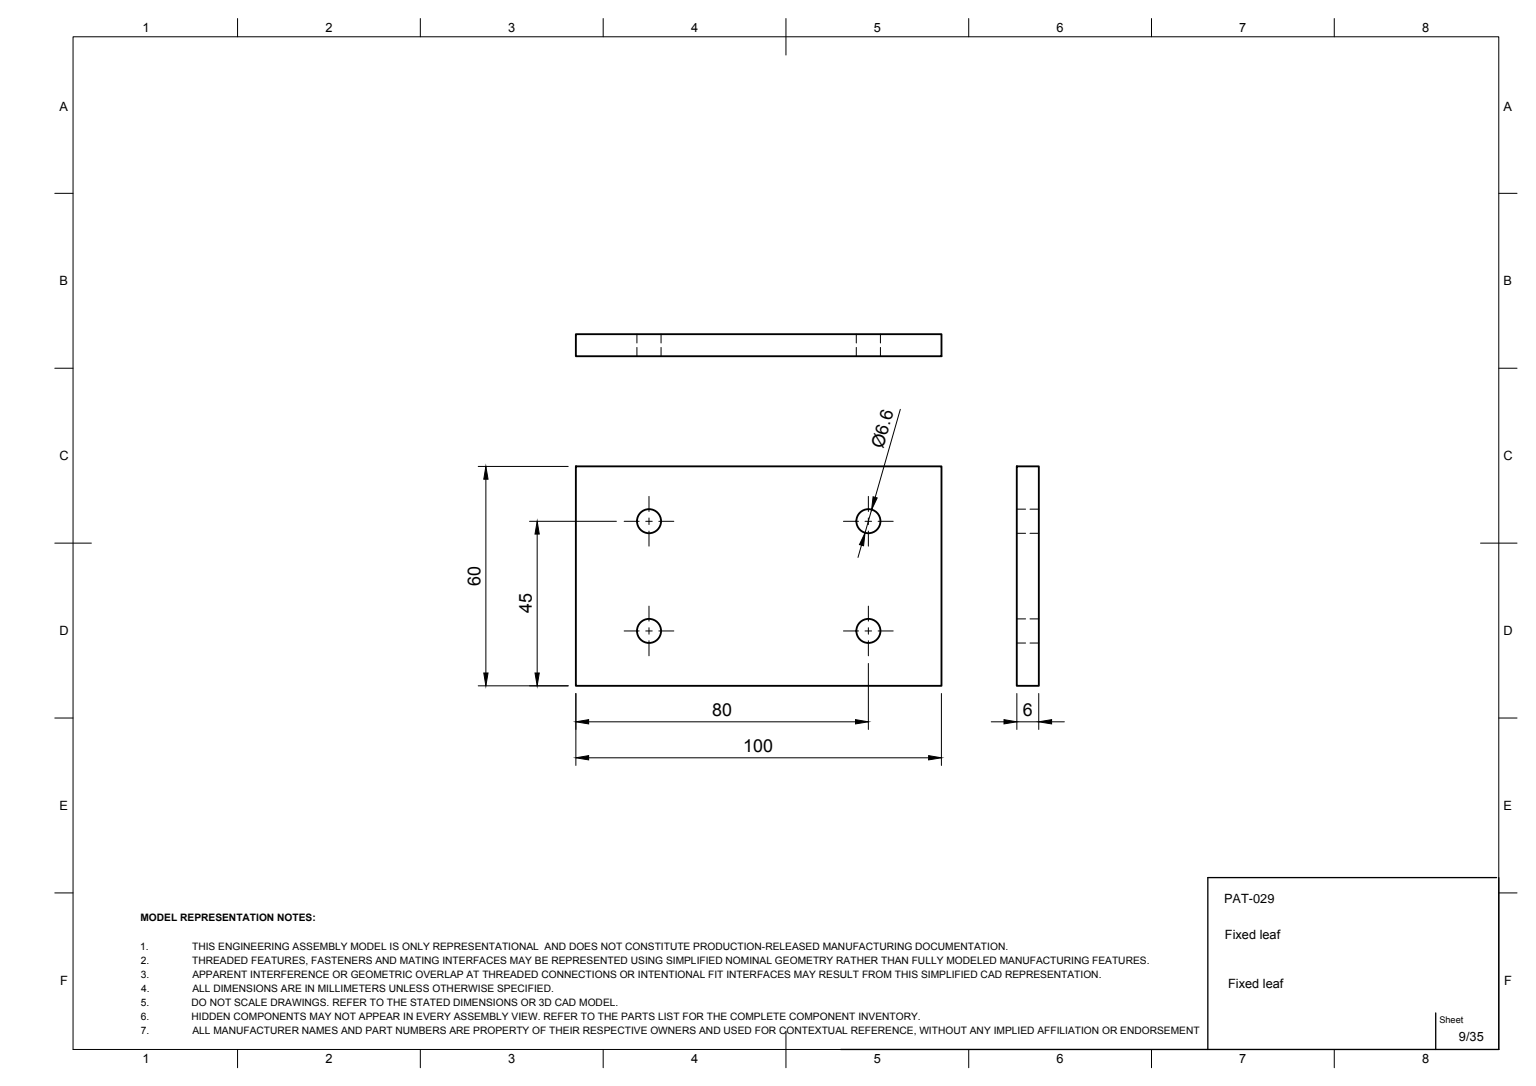
ISO-10303-21;
HEADER;
/* Generated by software containing ST-Developer
 * from STEP Tools, Inc. (www.steptools.com) 
 */

FILE_DESCRIPTION(
/* description */ ('Door-style hinge test fixture with detent'),
/* implementation_level */ '2;1');

FILE_NAME(
/* name */ 'Fixed leaf.step',
/* time_stamp */ '2026-10-28T03:24:57-07:00',
/* author */ (''),
/* organization */ (''),
/* preprocessor_version */ 'ST-DEVELOPER v20.2',
/* originating_system */ 'Autodesk Translation Framework v15.17.0.0',
/* authorisation */ '');

FILE_SCHEMA (('AUTOMOTIVE_DESIGN { 1 0 10303 214 3 1 1 }'));
ENDSEC;

DATA;
#10=MECHANICAL_DESIGN_GEOMETRIC_PRESENTATION_REPRESENTATION('',(#327),#9813);
#264=SHAPE_REPRESENTATION_RELATIONSHIP('SRR','None',#9941,#295);
#295=ADVANCED_BREP_SHAPE_REPRESENTATION('',(#367),#9784);
#327=STYLED_ITEM('',(#10176),#367);
#367=MANIFOLD_SOLID_BREP('Body1',#4758);
#415=FACE_BOUND('',#1007,.T.);
#416=FACE_BOUND('',#1008,.T.);
#417=FACE_BOUND('',#1009,.T.);
#418=FACE_BOUND('',#1010,.T.);
#419=FACE_BOUND('',#1013,.T.);
#420=FACE_BOUND('',#1014,.T.);
#421=FACE_BOUND('',#1015,.T.);
#422=FACE_BOUND('',#1016,.T.);
#530=PLANE('',#5211);
#531=PLANE('',#5212);
#532=PLANE('',#5213);
#533=PLANE('',#5214);
#534=PLANE('',#5215);
#535=PLANE('',#5216);
#701=FACE_OUTER_BOUND('',#1002,.T.);
#702=FACE_OUTER_BOUND('',#1003,.T.);
#703=FACE_OUTER_BOUND('',#1004,.T.);
#704=FACE_OUTER_BOUND('',#1005,.T.);
#705=FACE_OUTER_BOUND('',#1006,.T.);
#706=FACE_OUTER_BOUND('',#1011,.T.);
#707=FACE_OUTER_BOUND('',#1012,.T.);
#708=FACE_OUTER_BOUND('',#1017,.T.);
#709=FACE_OUTER_BOUND('',#1018,.T.);
#710=FACE_OUTER_BOUND('',#1019,.T.);
#1002=EDGE_LOOP('',(#3375,#3376,#3377,#3378));
#1003=EDGE_LOOP('',(#3379,#3380,#3381,#3382));
#1004=EDGE_LOOP('',(#3383,#3384,#3385,#3386));
#1005=EDGE_LOOP('',(#3387,#3388,#3389,#3390));
#1006=EDGE_LOOP('',(#3391,#3392,#3393,#3394));
#1007=EDGE_LOOP('',(#3395));
#1008=EDGE_LOOP('',(#3396));
#1009=EDGE_LOOP('',(#3397));
#1010=EDGE_LOOP('',(#3398));
#1011=EDGE_LOOP('',(#3399,#3400,#3401,#3402));
#1012=EDGE_LOOP('',(#3403,#3404,#3405,#3406));
#1013=EDGE_LOOP('',(#3407));
#1014=EDGE_LOOP('',(#3408));
#1015=EDGE_LOOP('',(#3409));
#1016=EDGE_LOOP('',(#3410));
#1017=EDGE_LOOP('',(#3411,#3412,#3413,#3414));
#1018=EDGE_LOOP('',(#3415,#3416,#3417,#3418));
#1019=EDGE_LOOP('',(#3419,#3420,#3421,#3422));
#1402=LINE('',#7486,#1722);
#1403=LINE('',#7492,#1723);
#1404=LINE('',#7498,#1724);
#1405=LINE('',#7504,#1725);
#1406=LINE('',#7509,#1726);
#1407=LINE('',#7511,#1727);
#1408=LINE('',#7513,#1728);
#1409=LINE('',#7514,#1729);
#1410=LINE('',#7517,#1730);
#1411=LINE('',#7519,#1731);
#1412=LINE('',#7520,#1732);
#1413=LINE('',#7523,#1733);
#1414=LINE('',#7525,#1734);
#1415=LINE('',#7526,#1735);
#1416=LINE('',#7528,#1736);
#1417=LINE('',#7529,#1737);
#1722=VECTOR('',#5945,0.33);
#1723=VECTOR('',#5952,0.33);
#1724=VECTOR('',#5959,0.33);
#1725=VECTOR('',#5966,0.33);
#1726=VECTOR('',#5971,1.);
#1727=VECTOR('',#5972,1.);
#1728=VECTOR('',#5973,1.);
#1729=VECTOR('',#5974,1.);
#1730=VECTOR('',#5977,1.);
#1731=VECTOR('',#5978,1.);
#1732=VECTOR('',#5979,1.);
#1733=VECTOR('',#5982,1.);
#1734=VECTOR('',#5983,1.);
#1735=VECTOR('',#5984,1.);
#1736=VECTOR('',#5987,1.);
#1737=VECTOR('',#5988,1.);
#1990=CIRCLE('',#5200,0.33);
#1991=CIRCLE('',#5201,0.33);
#1992=CIRCLE('',#5203,0.33);
#1993=CIRCLE('',#5204,0.33);
#1994=CIRCLE('',#5206,0.33);
#1995=CIRCLE('',#5207,0.33);
#1996=CIRCLE('',#5209,0.33);
#1997=CIRCLE('',#5210,0.33);
#2277=VERTEX_POINT('',#7483);
#2278=VERTEX_POINT('',#7485);
#2279=VERTEX_POINT('',#7489);
#2280=VERTEX_POINT('',#7491);
#2281=VERTEX_POINT('',#7495);
#2282=VERTEX_POINT('',#7497);
#2283=VERTEX_POINT('',#7501);
#2284=VERTEX_POINT('',#7503);
#2285=VERTEX_POINT('',#7507);
#2286=VERTEX_POINT('',#7508);
#2287=VERTEX_POINT('',#7510);
#2288=VERTEX_POINT('',#7512);
#2289=VERTEX_POINT('',#7516);
#2290=VERTEX_POINT('',#7518);
#2291=VERTEX_POINT('',#7522);
#2292=VERTEX_POINT('',#7524);
#2704=EDGE_CURVE('',#2277,#2277,#1990,.T.);
#2705=EDGE_CURVE('',#2277,#2278,#1402,.T.);
#2706=EDGE_CURVE('',#2278,#2278,#1991,.T.);
#2707=EDGE_CURVE('',#2279,#2279,#1992,.T.);
#2708=EDGE_CURVE('',#2279,#2280,#1403,.T.);
#2709=EDGE_CURVE('',#2280,#2280,#1993,.T.);
#2710=EDGE_CURVE('',#2281,#2281,#1994,.T.);
#2711=EDGE_CURVE('',#2281,#2282,#1404,.T.);
#2712=EDGE_CURVE('',#2282,#2282,#1995,.T.);
#2713=EDGE_CURVE('',#2283,#2283,#1996,.T.);
#2714=EDGE_CURVE('',#2283,#2284,#1405,.T.);
#2715=EDGE_CURVE('',#2284,#2284,#1997,.T.);
#2716=EDGE_CURVE('',#2285,#2286,#1406,.T.);
#2717=EDGE_CURVE('',#2286,#2287,#1407,.T.);
#2718=EDGE_CURVE('',#2288,#2287,#1408,.T.);
#2719=EDGE_CURVE('',#2285,#2288,#1409,.T.);
#2720=EDGE_CURVE('',#2289,#2285,#1410,.T.);
#2721=EDGE_CURVE('',#2290,#2288,#1411,.T.);
#2722=EDGE_CURVE('',#2289,#2290,#1412,.T.);
#2723=EDGE_CURVE('',#2291,#2289,#1413,.T.);
#2724=EDGE_CURVE('',#2292,#2290,#1414,.T.);
#2725=EDGE_CURVE('',#2291,#2292,#1415,.T.);
#2726=EDGE_CURVE('',#2286,#2291,#1416,.T.);
#2727=EDGE_CURVE('',#2287,#2292,#1417,.T.);
#3375=ORIENTED_EDGE('',*,*,#2704,.F.);
#3376=ORIENTED_EDGE('',*,*,#2705,.T.);
#3377=ORIENTED_EDGE('',*,*,#2706,.F.);
#3378=ORIENTED_EDGE('',*,*,#2705,.F.);
#3379=ORIENTED_EDGE('',*,*,#2707,.F.);
#3380=ORIENTED_EDGE('',*,*,#2708,.T.);
#3381=ORIENTED_EDGE('',*,*,#2709,.F.);
#3382=ORIENTED_EDGE('',*,*,#2708,.F.);
#3383=ORIENTED_EDGE('',*,*,#2710,.F.);
#3384=ORIENTED_EDGE('',*,*,#2711,.T.);
#3385=ORIENTED_EDGE('',*,*,#2712,.F.);
#3386=ORIENTED_EDGE('',*,*,#2711,.F.);
#3387=ORIENTED_EDGE('',*,*,#2713,.F.);
#3388=ORIENTED_EDGE('',*,*,#2714,.T.);
#3389=ORIENTED_EDGE('',*,*,#2715,.F.);
#3390=ORIENTED_EDGE('',*,*,#2714,.F.);
#3391=ORIENTED_EDGE('',*,*,#2716,.T.);
#3392=ORIENTED_EDGE('',*,*,#2717,.T.);
#3393=ORIENTED_EDGE('',*,*,#2718,.F.);
#3394=ORIENTED_EDGE('',*,*,#2719,.F.);
#3395=ORIENTED_EDGE('',*,*,#2706,.T.);
#3396=ORIENTED_EDGE('',*,*,#2709,.T.);
#3397=ORIENTED_EDGE('',*,*,#2712,.T.);
#3398=ORIENTED_EDGE('',*,*,#2715,.T.);
#3399=ORIENTED_EDGE('',*,*,#2720,.T.);
#3400=ORIENTED_EDGE('',*,*,#2719,.T.);
#3401=ORIENTED_EDGE('',*,*,#2721,.F.);
#3402=ORIENTED_EDGE('',*,*,#2722,.F.);
#3403=ORIENTED_EDGE('',*,*,#2723,.T.);
#3404=ORIENTED_EDGE('',*,*,#2722,.T.);
#3405=ORIENTED_EDGE('',*,*,#2724,.F.);
#3406=ORIENTED_EDGE('',*,*,#2725,.F.);
#3407=ORIENTED_EDGE('',*,*,#2704,.T.);
#3408=ORIENTED_EDGE('',*,*,#2707,.T.);
#3409=ORIENTED_EDGE('',*,*,#2710,.T.);
#3410=ORIENTED_EDGE('',*,*,#2713,.T.);
#3411=ORIENTED_EDGE('',*,*,#2726,.T.);
#3412=ORIENTED_EDGE('',*,*,#2725,.T.);
#3413=ORIENTED_EDGE('',*,*,#2727,.F.);
#3414=ORIENTED_EDGE('',*,*,#2717,.F.);
#3415=ORIENTED_EDGE('',*,*,#2727,.T.);
#3416=ORIENTED_EDGE('',*,*,#2724,.T.);
#3417=ORIENTED_EDGE('',*,*,#2721,.T.);
#3418=ORIENTED_EDGE('',*,*,#2718,.T.);
#3419=ORIENTED_EDGE('',*,*,#2726,.F.);
#3420=ORIENTED_EDGE('',*,*,#2716,.F.);
#3421=ORIENTED_EDGE('',*,*,#2720,.F.);
#3422=ORIENTED_EDGE('',*,*,#2723,.F.);
#4389=CYLINDRICAL_SURFACE('',#5199,0.33);
#4390=CYLINDRICAL_SURFACE('',#5202,0.33);
#4391=CYLINDRICAL_SURFACE('',#5205,0.33);
#4392=CYLINDRICAL_SURFACE('',#5208,0.33);
#4506=ADVANCED_FACE('',(#701),#4389,.F.);
#4507=ADVANCED_FACE('',(#702),#4390,.F.);
#4508=ADVANCED_FACE('',(#703),#4391,.F.);
#4509=ADVANCED_FACE('',(#704),#4392,.F.);
#4510=ADVANCED_FACE('',(#705,#415,#416,#417,#418),#530,.T.);
#4511=ADVANCED_FACE('',(#706),#531,.T.);
#4512=ADVANCED_FACE('',(#707,#419,#420,#421,#422),#532,.T.);
#4513=ADVANCED_FACE('',(#708),#533,.T.);
#4514=ADVANCED_FACE('',(#709),#534,.T.);
#4515=ADVANCED_FACE('',(#710),#535,.F.);
#4758=CLOSED_SHELL('',(#4506,#4507,#4508,#4509,#4510,#4511,#4512,#4513,
#4514,#4515));
#5198=AXIS2_PLACEMENT_3D('',#7481,#5939,#5940);
#5199=AXIS2_PLACEMENT_3D('',#7482,#5941,#5942);
#5200=AXIS2_PLACEMENT_3D('',#7484,#5943,#5944);
#5201=AXIS2_PLACEMENT_3D('',#7487,#5946,#5947);
#5202=AXIS2_PLACEMENT_3D('',#7488,#5948,#5949);
#5203=AXIS2_PLACEMENT_3D('',#7490,#5950,#5951);
#5204=AXIS2_PLACEMENT_3D('',#7493,#5953,#5954);
#5205=AXIS2_PLACEMENT_3D('',#7494,#5955,#5956);
#5206=AXIS2_PLACEMENT_3D('',#7496,#5957,#5958);
#5207=AXIS2_PLACEMENT_3D('',#7499,#5960,#5961);
#5208=AXIS2_PLACEMENT_3D('',#7500,#5962,#5963);
#5209=AXIS2_PLACEMENT_3D('',#7502,#5964,#5965);
#5210=AXIS2_PLACEMENT_3D('',#7505,#5967,#5968);
#5211=AXIS2_PLACEMENT_3D('',#7506,#5969,#5970);
#5212=AXIS2_PLACEMENT_3D('',#7515,#5975,#5976);
#5213=AXIS2_PLACEMENT_3D('',#7521,#5980,#5981);
#5214=AXIS2_PLACEMENT_3D('',#7527,#5985,#5986);
#5215=AXIS2_PLACEMENT_3D('',#7530,#5989,#5990);
#5216=AXIS2_PLACEMENT_3D('',#7531,#5991,#5992);
#5939=DIRECTION('axis',(0.,0.,1.));
#5940=DIRECTION('refdir',(1.,0.,0.));
#5941=DIRECTION('center_axis',(0.,1.,0.));
#5942=DIRECTION('ref_axis',(1.,0.,0.));
#5943=DIRECTION('center_axis',(0.,1.,0.));
#5944=DIRECTION('ref_axis',(1.,0.,0.));
#5945=DIRECTION('',(0.,1.,0.));
#5946=DIRECTION('center_axis',(0.,-1.,0.));
#5947=DIRECTION('ref_axis',(1.,0.,0.));
#5948=DIRECTION('center_axis',(0.,1.,0.));
#5949=DIRECTION('ref_axis',(1.,0.,0.));
#5950=DIRECTION('center_axis',(0.,1.,0.));
#5951=DIRECTION('ref_axis',(1.,0.,0.));
#5952=DIRECTION('',(0.,1.,0.));
#5953=DIRECTION('center_axis',(0.,-1.,0.));
#5954=DIRECTION('ref_axis',(1.,0.,0.));
#5955=DIRECTION('center_axis',(0.,1.,0.));
#5956=DIRECTION('ref_axis',(1.,0.,0.));
#5957=DIRECTION('center_axis',(0.,1.,0.));
#5958=DIRECTION('ref_axis',(1.,0.,0.));
#5959=DIRECTION('',(0.,1.,0.));
#5960=DIRECTION('center_axis',(0.,-1.,0.));
#5961=DIRECTION('ref_axis',(1.,0.,0.));
#5962=DIRECTION('center_axis',(0.,1.,0.));
#5963=DIRECTION('ref_axis',(1.,0.,0.));
#5964=DIRECTION('center_axis',(0.,1.,0.));
#5965=DIRECTION('ref_axis',(1.,0.,0.));
#5966=DIRECTION('',(0.,1.,0.));
#5967=DIRECTION('center_axis',(0.,-1.,0.));
#5968=DIRECTION('ref_axis',(1.,0.,0.));
#5969=DIRECTION('center_axis',(0.,1.,0.));
#5970=DIRECTION('ref_axis',(-1.,0.,0.));
#5971=DIRECTION('',(-1.,0.,0.));
#5972=DIRECTION('',(0.,0.,1.));
#5973=DIRECTION('',(-1.,0.,0.));
#5974=DIRECTION('',(0.,0.,1.));
#5975=DIRECTION('center_axis',(1.,0.,0.));
#5976=DIRECTION('ref_axis',(0.,1.,0.));
#5977=DIRECTION('',(0.,1.,0.));
#5978=DIRECTION('',(0.,1.,0.));
#5979=DIRECTION('',(0.,0.,1.));
#5980=DIRECTION('center_axis',(0.,-1.,0.));
#5981=DIRECTION('ref_axis',(1.,0.,0.));
#5982=DIRECTION('',(1.,0.,0.));
#5983=DIRECTION('',(1.,0.,0.));
#5984=DIRECTION('',(0.,0.,1.));
#5985=DIRECTION('center_axis',(-1.,0.,0.));
#5986=DIRECTION('ref_axis',(0.,-1.,0.));
#5987=DIRECTION('',(0.,-1.,0.));
#5988=DIRECTION('',(0.,-1.,0.));
#5989=DIRECTION('center_axis',(0.,0.,1.));
#5990=DIRECTION('ref_axis',(1.,0.,0.));
#5991=DIRECTION('center_axis',(0.,0.,1.));
#5992=DIRECTION('ref_axis',(1.,0.,0.));
#7481=CARTESIAN_POINT('',(0.,0.,0.));
#7482=CARTESIAN_POINT('Origin',(-6.5,-0.4,5.5));
#7483=CARTESIAN_POINT('',(-6.83,-0.3,5.5));
#7484=CARTESIAN_POINT('Origin',(-6.5,-0.3,5.5));
#7485=CARTESIAN_POINT('',(-6.83,0.3,5.5));
#7486=CARTESIAN_POINT('',(-6.83,-0.4,5.5));
#7487=CARTESIAN_POINT('Origin',(-6.5,0.3,5.5));
#7488=CARTESIAN_POINT('Origin',(-12.5,-0.4,8.5));
#7489=CARTESIAN_POINT('',(-12.83,-0.3,8.5));
#7490=CARTESIAN_POINT('Origin',(-12.5,-0.3,8.5));
#7491=CARTESIAN_POINT('',(-12.83,0.3,8.5));
#7492=CARTESIAN_POINT('',(-12.83,-0.4,8.5));
#7493=CARTESIAN_POINT('Origin',(-12.5,0.3,8.5));
#7494=CARTESIAN_POINT('Origin',(-12.5,-0.4,5.5));
#7495=CARTESIAN_POINT('',(-12.83,-0.3,5.5));
#7496=CARTESIAN_POINT('Origin',(-12.5,-0.3,5.5));
#7497=CARTESIAN_POINT('',(-12.83,0.3,5.5));
#7498=CARTESIAN_POINT('',(-12.83,-0.4,5.5));
#7499=CARTESIAN_POINT('Origin',(-12.5,0.3,5.5));
#7500=CARTESIAN_POINT('Origin',(-6.5,-0.4,8.5));
#7501=CARTESIAN_POINT('',(-6.83,-0.3,8.5));
#7502=CARTESIAN_POINT('Origin',(-6.5,-0.3,8.5));
#7503=CARTESIAN_POINT('',(-6.83,0.3,8.5));
#7504=CARTESIAN_POINT('',(-6.83,-0.4,8.5));
#7505=CARTESIAN_POINT('Origin',(-6.5,0.3,8.5));
#7506=CARTESIAN_POINT('Origin',(-4.5,0.3,4.));
#7507=CARTESIAN_POINT('',(-4.5,0.3,4.));
#7508=CARTESIAN_POINT('',(-14.5,0.3,4.));
#7509=CARTESIAN_POINT('',(-4.5,0.3,4.));
#7510=CARTESIAN_POINT('',(-14.5,0.3,10.));
#7511=CARTESIAN_POINT('',(-14.5,0.3,4.));
#7512=CARTESIAN_POINT('',(-4.5,0.3,10.));
#7513=CARTESIAN_POINT('',(-4.5,0.3,10.));
#7514=CARTESIAN_POINT('',(-4.5,0.3,4.));
#7515=CARTESIAN_POINT('Origin',(-4.5,-0.3,4.));
#7516=CARTESIAN_POINT('',(-4.5,-0.3,4.));
#7517=CARTESIAN_POINT('',(-4.5,-0.3,4.));
#7518=CARTESIAN_POINT('',(-4.5,-0.3,10.));
#7519=CARTESIAN_POINT('',(-4.5,-0.3,10.));
#7520=CARTESIAN_POINT('',(-4.5,-0.3,4.));
#7521=CARTESIAN_POINT('Origin',(-14.5,-0.3,4.));
#7522=CARTESIAN_POINT('',(-14.5,-0.3,4.));
#7523=CARTESIAN_POINT('',(-14.5,-0.3,4.));
#7524=CARTESIAN_POINT('',(-14.5,-0.3,10.));
#7525=CARTESIAN_POINT('',(-14.5,-0.3,10.));
#7526=CARTESIAN_POINT('',(-14.5,-0.3,4.));
#7527=CARTESIAN_POINT('Origin',(-14.5,0.3,4.));
#7528=CARTESIAN_POINT('',(-14.5,0.3,4.));
#7529=CARTESIAN_POINT('',(-14.5,0.3,10.));
#7530=CARTESIAN_POINT('Origin',(-9.5,0.,10.));
#7531=CARTESIAN_POINT('Origin',(-9.5,0.,4.));
#9748=UNCERTAINTY_MEASURE_WITH_UNIT(LENGTH_MEASURE(0.001),#9814,
'DISTANCE_ACCURACY_VALUE',
'Maximum model space distance between geometric entities at asserted c
onnectivities');
#9777=UNCERTAINTY_MEASURE_WITH_UNIT(LENGTH_MEASURE(0.001),#9814,
'DISTANCE_ACCURACY_VALUE',
'Maximum model space distance between geometric entities at asserted c
onnectivities');
#9784=(
GEOMETRIC_REPRESENTATION_CONTEXT(3)
GLOBAL_UNCERTAINTY_ASSIGNED_CONTEXT((#9748))
GLOBAL_UNIT_ASSIGNED_CONTEXT((#9814,#9816,#9817))
REPRESENTATION_CONTEXT('','3D')
);
#9813=(
GEOMETRIC_REPRESENTATION_CONTEXT(3)
GLOBAL_UNCERTAINTY_ASSIGNED_CONTEXT((#9777))
GLOBAL_UNIT_ASSIGNED_CONTEXT((#9814,#9816,#9817))
REPRESENTATION_CONTEXT('','3D')
);
#9814=(
LENGTH_UNIT()
NAMED_UNIT(*)
SI_UNIT(.CENTI.,.METRE.)
);
#9816=(
NAMED_UNIT(*)
PLANE_ANGLE_UNIT()
SI_UNIT($,.RADIAN.)
);
#9817=(
NAMED_UNIT(*)
SI_UNIT($,.STERADIAN.)
SOLID_ANGLE_UNIT()
);
#9824=SHAPE_DEFINITION_REPRESENTATION(#9859,#9941);
#9859=PRODUCT_DEFINITION_SHAPE('',$,#9977);
#9941=SHAPE_REPRESENTATION('',(#5198),#9784);
#9970=PRODUCT_DEFINITION_CONTEXT('part definition',#10077,'design');
#9977=PRODUCT_DEFINITION('Fixed leaf','Fixed leaf',#10012,#9970);
#10012=PRODUCT_DEFINITION_FORMATION('',$,#10085);
#10077=APPLICATION_CONTEXT(
'Core Data for Automotive Mechanical Design Process');
#10078=PRODUCT_CONTEXT('part definition',#10077,'mechanical');
#10085=PRODUCT('Fixed leaf','Fixed leaf','Fixed leaf',(#10078));
#10170=COLOUR_RGB('Sky Blue',0.24,0.69,0.87);
#10171=FILL_AREA_STYLE_COLOUR('',#10170);
#10172=FILL_AREA_STYLE('',(#10171));
#10173=SURFACE_STYLE_FILL_AREA(#10172);
#10174=SURFACE_SIDE_STYLE('',(#10173));
#10175=SURFACE_STYLE_USAGE(.BOTH.,#10174);
#10176=PRESENTATION_STYLE_ASSIGNMENT((#10175));
ENDSEC;
END-ISO-10303-21;
